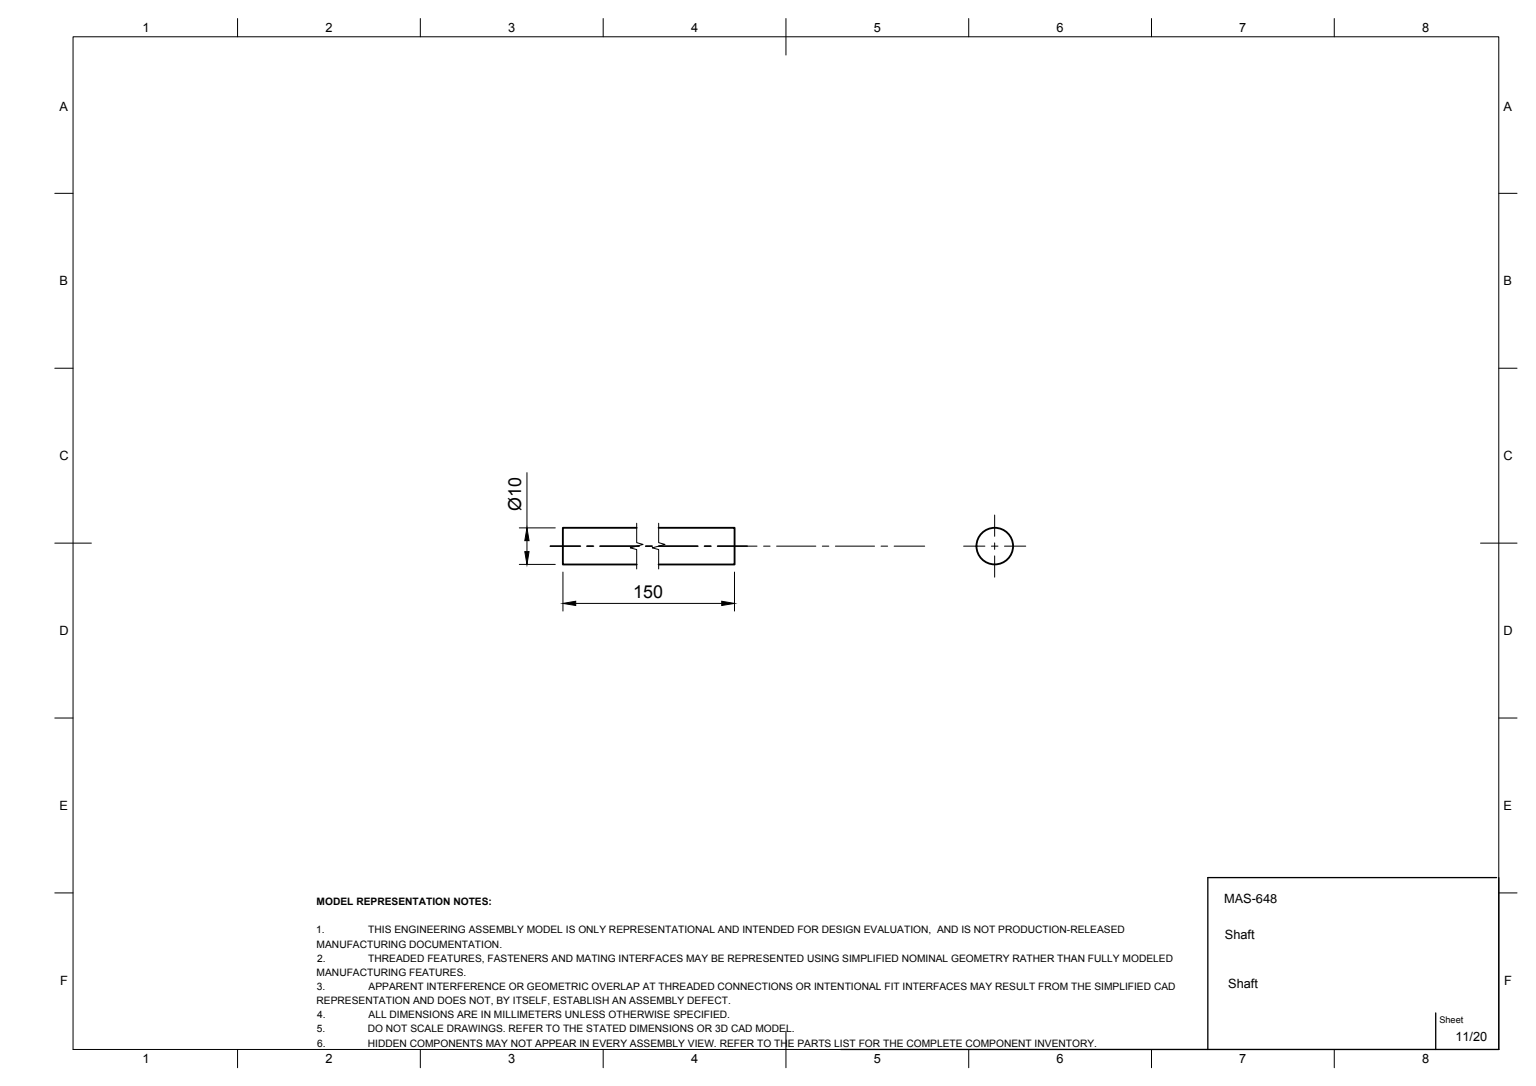
ISO-10303-21;
HEADER;
FILE_DESCRIPTION((''),'2;1');
FILE_NAME('Shaft.step','2026-10-09T12:47:58-07:00',(''),(''),'','','');
FILE_SCHEMA (('AUTOMOTIVE_DESIGN { 1 0 10303 214 3 1 1 }'));
ENDSEC;
DATA;
#10=MECHANICAL_DESIGN_GEOMETRIC_PRESENTATION_REPRESENTATION('',(#314),#3475);
#176=CIRCLE('',#2025,5.) ;
#177=CIRCLE('',#2026,5.) ;
#262=CYLINDRICAL_SURFACE('',#2024,5.) ;
#290=SHAPE_REPRESENTATION_RELATIONSHIP('SRR','None',#3545,#302) ;
#302=ADVANCED_BREP_SHAPE_REPRESENTATION('',(#326),#3465) ;
#314=STYLED_ITEM('',(#3628),#326) ;
#326=MANIFOLD_SOLID_BREP('Body1',#1828) ;
#367=FACE_OUTER_BOUND('',#488,.T.) ;
#368=FACE_OUTER_BOUND('',#489,.T.) ;
#369=FACE_OUTER_BOUND('',#490,.T.) ;
#488=EDGE_LOOP('',(#1346,#1347,#1348,#1349)) ;
#489=EDGE_LOOP('',(#1350)) ;
#490=EDGE_LOOP('',(#1351)) ;
#649=LINE('',#3067,#768) ;
#768=VECTOR('',#2390,5.) ;
#875=VERTEX_POINT('',#3064) ;
#876=VERTEX_POINT('',#3066) ;
#1045=EDGE_CURVE('',#875,#875,#176,.T.) ;
#1046=EDGE_CURVE('',#875,#876,#649,.T.) ;
#1047=EDGE_CURVE('',#876,#876,#177,.T.) ;
#1346=ORIENTED_EDGE('',*,*,#1045,.T.) ;
#1347=ORIENTED_EDGE('',*,*,#1046,.T.) ;
#1348=ORIENTED_EDGE('',*,*,#1047,.F.) ;
#1349=ORIENTED_EDGE('',*,*,#1046,.F.) ;
#1350=ORIENTED_EDGE('',*,*,#1047,.T.) ;
#1351=ORIENTED_EDGE('',*,*,#1045,.F.) ;
#1670=PLANE('',#2027) ;
#1671=PLANE('',#2028) ;
#1743=ADVANCED_FACE('',(#367),#262,.T.) ;
#1744=ADVANCED_FACE('',(#368),#1670,.T.) ;
#1745=ADVANCED_FACE('',(#369),#1671,.F.) ;
#1828=CLOSED_SHELL('',(#1743,#1744,#1745)) ;
#2023=AXIS2_PLACEMENT_3D('',#3062,#2384,#2385) ;
#2024=AXIS2_PLACEMENT_3D('',#3063,#2386,#2387) ;
#2025=AXIS2_PLACEMENT_3D('',#3065,#2388,#2389) ;
#2026=AXIS2_PLACEMENT_3D('',#3068,#2391,#2392) ;
#2027=AXIS2_PLACEMENT_3D('',#3069,#2393,#2394) ;
#2028=AXIS2_PLACEMENT_3D('',#3070,#2395,#2396) ;
#2384=DIRECTION('axis',(0.,0.,1.)) ;
#2385=DIRECTION('refdir',(1.,0.,0.)) ;
#2386=DIRECTION('center_axis',(0.,0.,-1.)) ;
#2387=DIRECTION('ref_axis',(-1.,0.,0.)) ;
#2388=DIRECTION('center_axis',(0.,0.,1.)) ;
#2389=DIRECTION('ref_axis',(1.,0.,0.)) ;
#2390=DIRECTION('',(0.,0.,1.)) ;
#2391=DIRECTION('center_axis',(0.,0.,1.)) ;
#2392=DIRECTION('ref_axis',(1.,0.,0.)) ;
#2393=DIRECTION('center_axis',(0.,0.,1.)) ;
#2394=DIRECTION('ref_axis',(1.,0.,0.)) ;
#2395=DIRECTION('center_axis',(0.,0.,1.)) ;
#2396=DIRECTION('ref_axis',(1.,0.,0.)) ;
#3062=CARTESIAN_POINT('',(0.,0.,0.)) ;
#3063=CARTESIAN_POINT('Origin',(0.,0.,150.)) ;
#3064=CARTESIAN_POINT('',(5.,-6.12323399573677E-16,0.)) ;
#3065=CARTESIAN_POINT('Origin',(0.,0.,0.)) ;
#3066=CARTESIAN_POINT('',(5.,-6.12323399573677E-16,150.)) ;
#3067=CARTESIAN_POINT('',(5.,-6.12323399573677E-16,150.)) ;
#3068=CARTESIAN_POINT('Origin',(0.,0.,150.)) ;
#3069=CARTESIAN_POINT('Origin',(0.,0.,150.)) ;
#3070=CARTESIAN_POINT('Origin',(0.,0.,0.)) ;
#3447=UNCERTAINTY_MEASURE_WITH_UNIT(LENGTH_MEASURE(0.01),#3476,
'DISTANCE_ACCURACY_VALUE',
'Maximum model space distance between geometric entities at asserted c
onnectivities') ;
#3457=UNCERTAINTY_MEASURE_WITH_UNIT(LENGTH_MEASURE(0.01),#3476,
'DISTANCE_ACCURACY_VALUE',
'Maximum model space distance between geometric entities at asserted c
onnectivities') ;
#3465=(
GEOMETRIC_REPRESENTATION_CONTEXT(3)
GLOBAL_UNCERTAINTY_ASSIGNED_CONTEXT((#3447))
GLOBAL_UNIT_ASSIGNED_CONTEXT((#3476,#3478,#3479))
REPRESENTATION_CONTEXT('','3D')
) ;
#3475=(
GEOMETRIC_REPRESENTATION_CONTEXT(3)
GLOBAL_UNCERTAINTY_ASSIGNED_CONTEXT((#3457))
GLOBAL_UNIT_ASSIGNED_CONTEXT((#3476,#3478,#3479))
REPRESENTATION_CONTEXT('','3D')
) ;
#3476=(
LENGTH_UNIT()
NAMED_UNIT(*)
SI_UNIT(.MILLI.,.METRE.)
) ;
#3478=(
NAMED_UNIT(*)
PLANE_ANGLE_UNIT()
SI_UNIT($,.RADIAN.)
) ;
#3479=(
NAMED_UNIT(*)
SI_UNIT($,.STERADIAN.)
SOLID_ANGLE_UNIT()
) ;
#3487=SHAPE_DEFINITION_REPRESENTATION(#3508,#3545) ;
#3508=PRODUCT_DEFINITION_SHAPE('',$,#3563) ;
#3545=SHAPE_REPRESENTATION('',(#2023),#3465) ;
#3555=PRODUCT_DEFINITION_CONTEXT('part definition',#3608,'design') ;
#3563=PRODUCT_DEFINITION('Shaft','Shaft',#3580,#3555) ;
#3580=PRODUCT_DEFINITION_FORMATION('',$,#3617) ;
#3608=APPLICATION_CONTEXT(
'Core Data for Automotive Mechanical Design Process') ;
#3609=PRODUCT_CONTEXT('part definition',#3608,'mechanical') ;
#3617=PRODUCT('Shaft',
'Shaft',$,(#3609)) ;
#3628=PRESENTATION_STYLE_ASSIGNMENT((#3630)) ;
#3630=SURFACE_STYLE_USAGE(.BOTH.,#3632) ;
#3632=SURFACE_SIDE_STYLE('',(#3634)) ;
#3634=SURFACE_STYLE_FILL_AREA(#3636) ;
#3636=FILL_AREA_STYLE('Opaque(202,209,238)',(#3638)) ;
#3638=FILL_AREA_STYLE_COLOUR('Opaque(202,209,238)',#3640) ;
#3640=COLOUR_RGB('Opaque(202,209,238)', 0.09019608, 0.27058824, 0.51372549) ;
ENDSEC;
END-ISO-10303-21;
